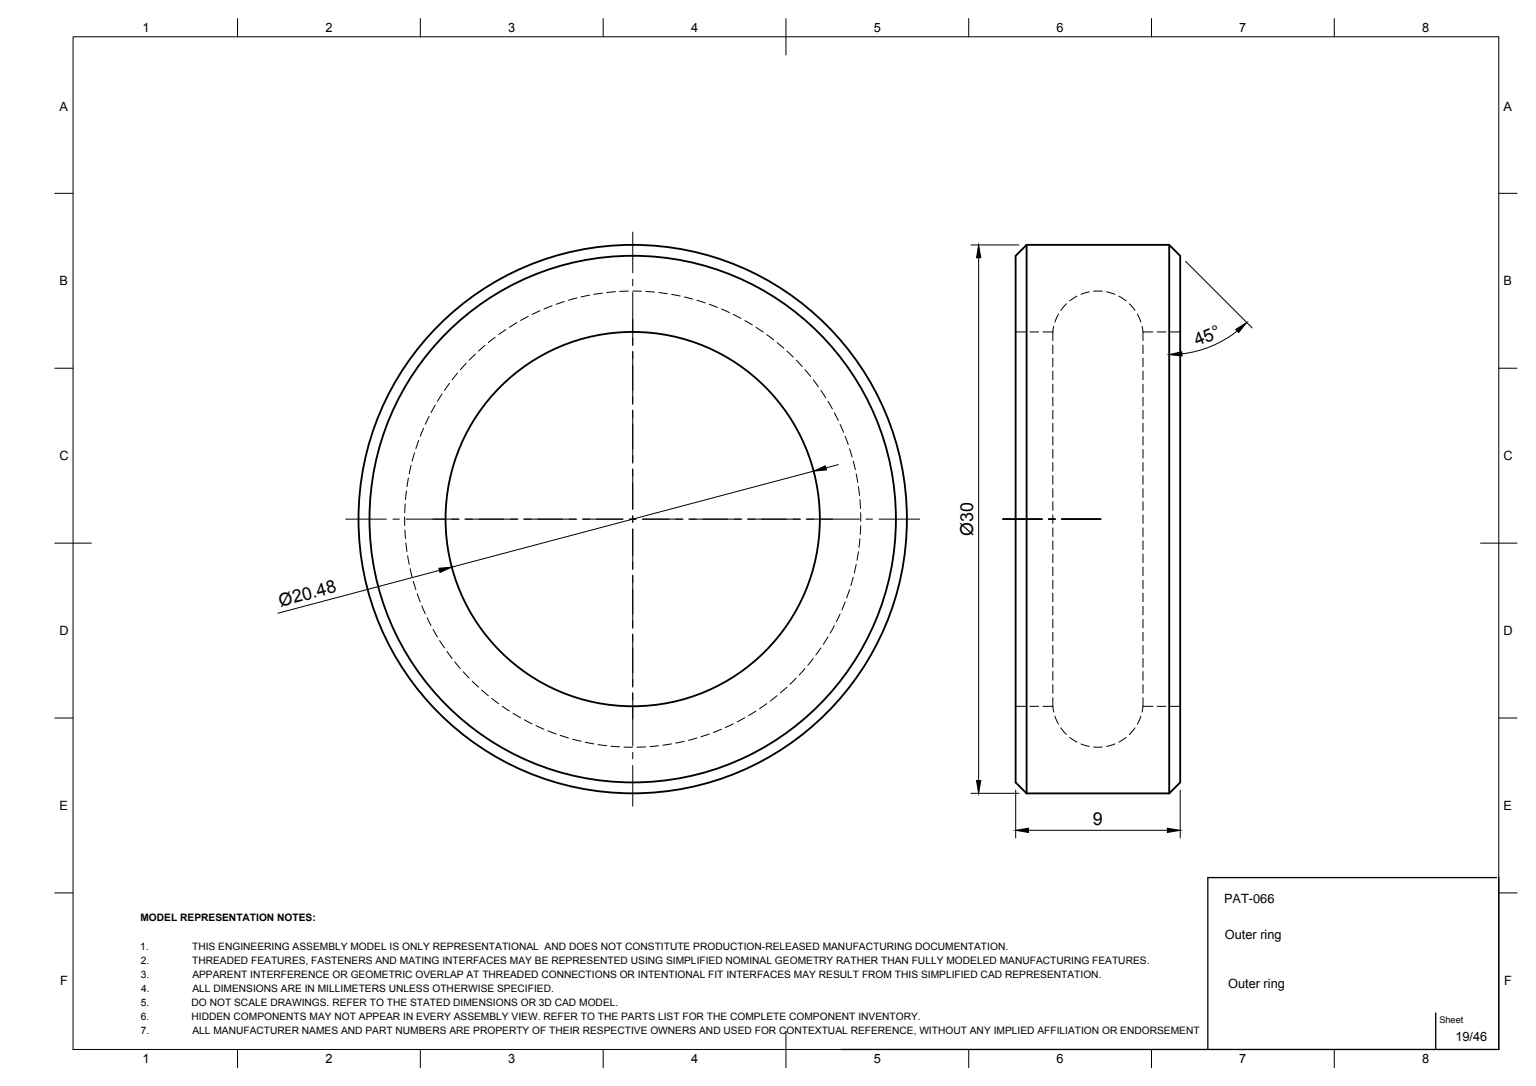
ISO-10303-21;
HEADER;
/* Generated by software containing ST-Developer
 * from STEP Tools, Inc. (www.steptools.com) 
 */

FILE_DESCRIPTION(
/* description */ ('Lever-operated bar clamp (toggle)'),
/* implementation_level */ '2;1');

FILE_NAME(
/* name */ 'Outer ring.step',
/* time_stamp */ '2026-10-28T03:25:02-07:00',
/* author */ (''),
/* organization */ (''),
/* preprocessor_version */ 'ST-DEVELOPER v20.2',
/* originating_system */ 'Autodesk Translation Framework v15.17.0.0',
/* authorisation */ '');

FILE_SCHEMA (('AUTOMOTIVE_DESIGN { 1 0 10303 214 3 1 1 }'));
ENDSEC;

DATA;
#10=MECHANICAL_DESIGN_GEOMETRIC_PRESENTATION_REPRESENTATION('',(#423),#12413);
#304=TOROIDAL_SURFACE('',#7349,1.,0.247676);
#310=CONICAL_SURFACE('',#7360,1.47,0.785398163397449);
#311=CONICAL_SURFACE('',#7364,1.47,0.785398163397449);
#347=SHAPE_REPRESENTATION_RELATIONSHIP('SRR','None',#12587,#385);
#385=ADVANCED_BREP_SHAPE_REPRESENTATION('',(#469),#12384);
#423=STYLED_ITEM('',(#12869),#469);
#469=MANIFOLD_SOLID_BREP('Body1',#6583);
#590=FACE_BOUND('',#1546,.T.);
#591=FACE_BOUND('',#1551,.T.);
#741=PLANE('',#7357);
#742=PLANE('',#7366);
#1047=FACE_OUTER_BOUND('',#1543,.T.);
#1048=FACE_OUTER_BOUND('',#1544,.T.);
#1049=FACE_OUTER_BOUND('',#1545,.T.);
#1050=FACE_OUTER_BOUND('',#1547,.T.);
#1051=FACE_OUTER_BOUND('',#1548,.T.);
#1052=FACE_OUTER_BOUND('',#1549,.T.);
#1053=FACE_OUTER_BOUND('',#1550,.T.);
#1054=FACE_OUTER_BOUND('',#1552,.T.);
#1543=EDGE_LOOP('',(#5077,#5078,#5079,#5080,#5081,#5082));
#1544=EDGE_LOOP('',(#5083,#5084,#5085,#5086,#5087));
#1545=EDGE_LOOP('',(#5088));
#1546=EDGE_LOOP('',(#5089));
#1547=EDGE_LOOP('',(#5090,#5091,#5092,#5093));
#1548=EDGE_LOOP('',(#5094,#5095,#5096,#5097));
#1549=EDGE_LOOP('',(#5098,#5099,#5100,#5101));
#1550=EDGE_LOOP('',(#5102));
#1551=EDGE_LOOP('',(#5103));
#1552=EDGE_LOOP('',(#5104,#5105,#5106,#5107,#5108));
#2045=LINE('',#10779,#2486);
#2046=LINE('',#10788,#2487);
#2047=LINE('',#10792,#2488);
#2048=LINE('',#10796,#2489);
#2049=LINE('',#10799,#2490);
#2486=VECTOR('',#8724,1.023815);
#2487=VECTOR('',#8735,1.47);
#2488=VECTOR('',#8740,1.5);
#2489=VECTOR('',#8745,1.47);
#2490=VECTOR('',#8750,1.023815);
#2867=CIRCLE('',#7350,1.023815);
#2868=CIRCLE('',#7351,1.023815);
#2869=CIRCLE('',#7352,0.247676);
#2870=CIRCLE('',#7353,1.023815);
#2871=CIRCLE('',#7354,1.023815);
#2872=CIRCLE('',#7356,1.023815);
#2873=CIRCLE('',#7358,1.44);
#2874=CIRCLE('',#7359,1.023815);
#2875=CIRCLE('',#7361,1.5);
#2876=CIRCLE('',#7363,1.5);
#2877=CIRCLE('',#7365,1.44);
#3291=VERTEX_POINT('',#10767);
#3292=VERTEX_POINT('',#10768);
#3293=VERTEX_POINT('',#10771);
#3294=VERTEX_POINT('',#10773);
#3295=VERTEX_POINT('',#10777);
#3296=VERTEX_POINT('',#10781);
#3297=VERTEX_POINT('',#10783);
#3298=VERTEX_POINT('',#10786);
#3299=VERTEX_POINT('',#10790);
#3300=VERTEX_POINT('',#10794);
#3943=EDGE_CURVE('',#3291,#3292,#2867,.T.);
#3944=EDGE_CURVE('',#3292,#3291,#2868,.T.);
#3945=EDGE_CURVE('',#3292,#3293,#2869,.T.);
#3946=EDGE_CURVE('',#3294,#3293,#2870,.T.);
#3947=EDGE_CURVE('',#3293,#3294,#2871,.T.);
#3948=EDGE_CURVE('',#3295,#3295,#2872,.T.);
#3949=EDGE_CURVE('',#3295,#3294,#2045,.T.);
#3950=EDGE_CURVE('',#3296,#3296,#2873,.T.);
#3951=EDGE_CURVE('',#3297,#3297,#2874,.T.);
#3952=EDGE_CURVE('',#3298,#3298,#2875,.T.);
#3953=EDGE_CURVE('',#3298,#3296,#2046,.T.);
#3954=EDGE_CURVE('',#3299,#3299,#2876,.T.);
#3955=EDGE_CURVE('',#3299,#3298,#2047,.T.);
#3956=EDGE_CURVE('',#3300,#3300,#2877,.T.);
#3957=EDGE_CURVE('',#3300,#3299,#2048,.T.);
#3958=EDGE_CURVE('',#3291,#3297,#2049,.T.);
#5077=ORIENTED_EDGE('',*,*,#3943,.F.);
#5078=ORIENTED_EDGE('',*,*,#3944,.F.);
#5079=ORIENTED_EDGE('',*,*,#3945,.T.);
#5080=ORIENTED_EDGE('',*,*,#3946,.F.);
#5081=ORIENTED_EDGE('',*,*,#3947,.F.);
#5082=ORIENTED_EDGE('',*,*,#3945,.F.);
#5083=ORIENTED_EDGE('',*,*,#3948,.T.);
#5084=ORIENTED_EDGE('',*,*,#3949,.T.);
#5085=ORIENTED_EDGE('',*,*,#3946,.T.);
#5086=ORIENTED_EDGE('',*,*,#3947,.T.);
#5087=ORIENTED_EDGE('',*,*,#3949,.F.);
#5088=ORIENTED_EDGE('',*,*,#3950,.F.);
#5089=ORIENTED_EDGE('',*,*,#3951,.T.);
#5090=ORIENTED_EDGE('',*,*,#3952,.F.);
#5091=ORIENTED_EDGE('',*,*,#3953,.T.);
#5092=ORIENTED_EDGE('',*,*,#3950,.T.);
#5093=ORIENTED_EDGE('',*,*,#3953,.F.);
#5094=ORIENTED_EDGE('',*,*,#3954,.F.);
#5095=ORIENTED_EDGE('',*,*,#3955,.T.);
#5096=ORIENTED_EDGE('',*,*,#3952,.T.);
#5097=ORIENTED_EDGE('',*,*,#3955,.F.);
#5098=ORIENTED_EDGE('',*,*,#3956,.F.);
#5099=ORIENTED_EDGE('',*,*,#3957,.T.);
#5100=ORIENTED_EDGE('',*,*,#3954,.T.);
#5101=ORIENTED_EDGE('',*,*,#3957,.F.);
#5102=ORIENTED_EDGE('',*,*,#3956,.T.);
#5103=ORIENTED_EDGE('',*,*,#3948,.F.);
#5104=ORIENTED_EDGE('',*,*,#3943,.T.);
#5105=ORIENTED_EDGE('',*,*,#3944,.T.);
#5106=ORIENTED_EDGE('',*,*,#3958,.T.);
#5107=ORIENTED_EDGE('',*,*,#3951,.F.);
#5108=ORIENTED_EDGE('',*,*,#3958,.F.);
#6096=CYLINDRICAL_SURFACE('',#7355,1.023815);
#6097=CYLINDRICAL_SURFACE('',#7362,1.5);
#6098=CYLINDRICAL_SURFACE('',#7367,1.023815);
#6322=ADVANCED_FACE('',(#1047),#304,.F.);
#6323=ADVANCED_FACE('',(#1048),#6096,.F.);
#6324=ADVANCED_FACE('',(#1049,#590),#741,.T.);
#6325=ADVANCED_FACE('',(#1050),#310,.T.);
#6326=ADVANCED_FACE('',(#1051),#6097,.T.);
#6327=ADVANCED_FACE('',(#1052),#311,.T.);
#6328=ADVANCED_FACE('',(#1053,#591),#742,.T.);
#6329=ADVANCED_FACE('',(#1054),#6098,.F.);
#6583=CLOSED_SHELL('',(#6322,#6323,#6324,#6325,#6326,#6327,#6328,#6329));
#7348=AXIS2_PLACEMENT_3D('',#10765,#8706,#8707);
#7349=AXIS2_PLACEMENT_3D('',#10766,#8708,#8709);
#7350=AXIS2_PLACEMENT_3D('',#10769,#8710,#8711);
#7351=AXIS2_PLACEMENT_3D('',#10770,#8712,#8713);
#7352=AXIS2_PLACEMENT_3D('',#10772,#8714,#8715);
#7353=AXIS2_PLACEMENT_3D('',#10774,#8716,#8717);
#7354=AXIS2_PLACEMENT_3D('',#10775,#8718,#8719);
#7355=AXIS2_PLACEMENT_3D('',#10776,#8720,#8721);
#7356=AXIS2_PLACEMENT_3D('',#10778,#8722,#8723);
#7357=AXIS2_PLACEMENT_3D('',#10780,#8725,#8726);
#7358=AXIS2_PLACEMENT_3D('',#10782,#8727,#8728);
#7359=AXIS2_PLACEMENT_3D('',#10784,#8729,#8730);
#7360=AXIS2_PLACEMENT_3D('',#10785,#8731,#8732);
#7361=AXIS2_PLACEMENT_3D('',#10787,#8733,#8734);
#7362=AXIS2_PLACEMENT_3D('',#10789,#8736,#8737);
#7363=AXIS2_PLACEMENT_3D('',#10791,#8738,#8739);
#7364=AXIS2_PLACEMENT_3D('',#10793,#8741,#8742);
#7365=AXIS2_PLACEMENT_3D('',#10795,#8743,#8744);
#7366=AXIS2_PLACEMENT_3D('',#10797,#8746,#8747);
#7367=AXIS2_PLACEMENT_3D('',#10798,#8748,#8749);
#8706=DIRECTION('axis',(0.,0.,1.));
#8707=DIRECTION('refdir',(1.,0.,0.));
#8708=DIRECTION('center_axis',(0.,-1.,0.));
#8709=DIRECTION('ref_axis',(0.,0.,-1.));
#8710=DIRECTION('center_axis',(0.,-1.,0.));
#8711=DIRECTION('ref_axis',(1.,0.,0.));
#8712=DIRECTION('center_axis',(0.,-1.,0.));
#8713=DIRECTION('ref_axis',(1.,0.,0.));
#8714=DIRECTION('center_axis',(1.,0.,1.22464679914735E-16));
#8715=DIRECTION('ref_axis',(-1.22464679914735E-16,0.,1.));
#8716=DIRECTION('center_axis',(0.,1.,0.));
#8717=DIRECTION('ref_axis',(1.,0.,0.));
#8718=DIRECTION('center_axis',(0.,1.,0.));
#8719=DIRECTION('ref_axis',(1.,0.,0.));
#8720=DIRECTION('center_axis',(0.,-1.,0.));
#8721=DIRECTION('ref_axis',(1.,0.,0.));
#8722=DIRECTION('center_axis',(0.,-1.,0.));
#8723=DIRECTION('ref_axis',(1.,0.,0.));
#8724=DIRECTION('',(0.,1.,0.));
#8725=DIRECTION('center_axis',(0.,1.,0.));
#8726=DIRECTION('ref_axis',(0.,0.,1.));
#8727=DIRECTION('center_axis',(0.,-1.,0.));
#8728=DIRECTION('ref_axis',(1.,0.,0.));
#8729=DIRECTION('center_axis',(0.,-1.,0.));
#8730=DIRECTION('ref_axis',(1.,0.,0.));
#8731=DIRECTION('center_axis',(0.,-1.,0.));
#8732=DIRECTION('ref_axis',(1.,0.,0.));
#8733=DIRECTION('center_axis',(0.,-1.,0.));
#8734=DIRECTION('ref_axis',(1.,0.,0.));
#8735=DIRECTION('',(0.707106781186548,0.707106781186547,8.65956056235494E-17));
#8736=DIRECTION('center_axis',(0.,-1.,0.));
#8737=DIRECTION('ref_axis',(1.,0.,0.));
#8738=DIRECTION('center_axis',(0.,-1.,0.));
#8739=DIRECTION('ref_axis',(1.,0.,0.));
#8740=DIRECTION('',(0.,1.,0.));
#8741=DIRECTION('center_axis',(0.,1.,0.));
#8742=DIRECTION('ref_axis',(1.,0.,0.));
#8743=DIRECTION('center_axis',(0.,-1.,0.));
#8744=DIRECTION('ref_axis',(1.,0.,0.));
#8745=DIRECTION('',(-0.707106781186548,0.707106781186547,-8.65956056235494E-17));
#8746=DIRECTION('center_axis',(0.,-1.,0.));
#8747=DIRECTION('ref_axis',(0.,0.,-1.));
#8748=DIRECTION('center_axis',(0.,-1.,0.));
#8749=DIRECTION('ref_axis',(1.,0.,0.));
#8750=DIRECTION('',(0.,1.,0.));
#10765=CARTESIAN_POINT('',(0.,0.,0.));
#10766=CARTESIAN_POINT('Origin',(0.,0.,0.));
#10767=CARTESIAN_POINT('',(-1.023815,0.246528389340863,-1.25381176266905E-16));
#10768=CARTESIAN_POINT('',(-1.25381176266905E-16,0.246528389340863,1.023815));
#10769=CARTESIAN_POINT('Origin',(0.,0.246528389340863,0.));
#10770=CARTESIAN_POINT('Origin',(0.,0.246528389340863,0.));
#10771=CARTESIAN_POINT('',(-1.25381176266905E-16,-0.246528389340863,1.023815));
#10772=CARTESIAN_POINT('Origin',(-1.22464679914735E-16,0.,1.));
#10773=CARTESIAN_POINT('',(-1.023815,-0.246528389340863,1.25381176266905E-16));
#10774=CARTESIAN_POINT('Origin',(0.,-0.246528389340863,0.));
#10775=CARTESIAN_POINT('Origin',(0.,-0.246528389340863,0.));
#10776=CARTESIAN_POINT('Origin',(0.,0.,0.));
#10777=CARTESIAN_POINT('',(-1.023815,-0.45,-1.25381176266905E-16));
#10778=CARTESIAN_POINT('Origin',(0.,-0.45,0.));
#10779=CARTESIAN_POINT('',(-1.023815,0.,-1.25381176266905E-16));
#10780=CARTESIAN_POINT('Origin',(1.44,0.45,0.));
#10781=CARTESIAN_POINT('',(-1.44,0.45,-1.76349139077219E-16));
#10782=CARTESIAN_POINT('Origin',(0.,0.45,0.));
#10783=CARTESIAN_POINT('',(-1.023815,0.45,-1.25381176266905E-16));
#10784=CARTESIAN_POINT('Origin',(0.,0.45,0.));
#10785=CARTESIAN_POINT('Origin',(0.,0.42,0.));
#10786=CARTESIAN_POINT('',(-1.5,0.39,-1.83697019872103E-16));
#10787=CARTESIAN_POINT('Origin',(0.,0.39,0.));
#10788=CARTESIAN_POINT('',(-1.47,0.42,-1.80023079474661E-16));
#10789=CARTESIAN_POINT('Origin',(0.,0.,0.));
#10790=CARTESIAN_POINT('',(-1.5,-0.39,-1.83697019872103E-16));
#10791=CARTESIAN_POINT('Origin',(0.,-0.39,0.));
#10792=CARTESIAN_POINT('',(-1.5,0.,-1.83697019872103E-16));
#10793=CARTESIAN_POINT('Origin',(0.,-0.42,0.));
#10794=CARTESIAN_POINT('',(-1.44,-0.45,-1.76349139077219E-16));
#10795=CARTESIAN_POINT('Origin',(0.,-0.45,0.));
#10796=CARTESIAN_POINT('',(-1.47,-0.42,-1.80023079474661E-16));
#10797=CARTESIAN_POINT('Origin',(1.023815,-0.45,0.));
#10798=CARTESIAN_POINT('Origin',(0.,0.,0.));
#10799=CARTESIAN_POINT('',(-1.023815,0.,-1.25381176266905E-16));
#12338=UNCERTAINTY_MEASURE_WITH_UNIT(LENGTH_MEASURE(0.001),#12414,
'DISTANCE_ACCURACY_VALUE',
'Maximum model space distance between geometric entities at asserted c
onnectivities');
#12367=UNCERTAINTY_MEASURE_WITH_UNIT(LENGTH_MEASURE(0.001),#12414,
'DISTANCE_ACCURACY_VALUE',
'Maximum model space distance between geometric entities at asserted c
onnectivities');
#12384=(
GEOMETRIC_REPRESENTATION_CONTEXT(3)
GLOBAL_UNCERTAINTY_ASSIGNED_CONTEXT((#12338))
GLOBAL_UNIT_ASSIGNED_CONTEXT((#12414,#12416,#12417))
REPRESENTATION_CONTEXT('','3D')
);
#12413=(
GEOMETRIC_REPRESENTATION_CONTEXT(3)
GLOBAL_UNCERTAINTY_ASSIGNED_CONTEXT((#12367))
GLOBAL_UNIT_ASSIGNED_CONTEXT((#12414,#12416,#12417))
REPRESENTATION_CONTEXT('','3D')
);
#12414=(
LENGTH_UNIT()
NAMED_UNIT(*)
SI_UNIT(.CENTI.,.METRE.)
);
#12416=(
NAMED_UNIT(*)
PLANE_ANGLE_UNIT()
SI_UNIT($,.RADIAN.)
);
#12417=(
NAMED_UNIT(*)
SI_UNIT($,.STERADIAN.)
SOLID_ANGLE_UNIT()
);
#12434=SHAPE_DEFINITION_REPRESENTATION(#12479,#12587);
#12479=PRODUCT_DEFINITION_SHAPE('',$,#12633);
#12587=SHAPE_REPRESENTATION('',(#7348),#12384);
#12616=PRODUCT_DEFINITION_CONTEXT('part definition',#12753,'design');
#12633=PRODUCT_DEFINITION('Outer ring','Outer ring',#12678,#12616);
#12678=PRODUCT_DEFINITION_FORMATION('',$,#12771);
#12753=APPLICATION_CONTEXT(
'Core Data for Automotive Mechanical Design Process');
#12754=PRODUCT_CONTEXT('part definition',#12753,'mechanical');
#12771=PRODUCT('Outer ring','Outer ring','Outer ring',(#12754));
#12863=COLOUR_RGB('Grey',0.48,0.52,0.57);
#12864=FILL_AREA_STYLE_COLOUR('',#12863);
#12865=FILL_AREA_STYLE('',(#12864));
#12866=SURFACE_STYLE_FILL_AREA(#12865);
#12867=SURFACE_SIDE_STYLE('',(#12866));
#12868=SURFACE_STYLE_USAGE(.BOTH.,#12867);
#12869=PRESENTATION_STYLE_ASSIGNMENT((#12868));
ENDSEC;
END-ISO-10303-21;
